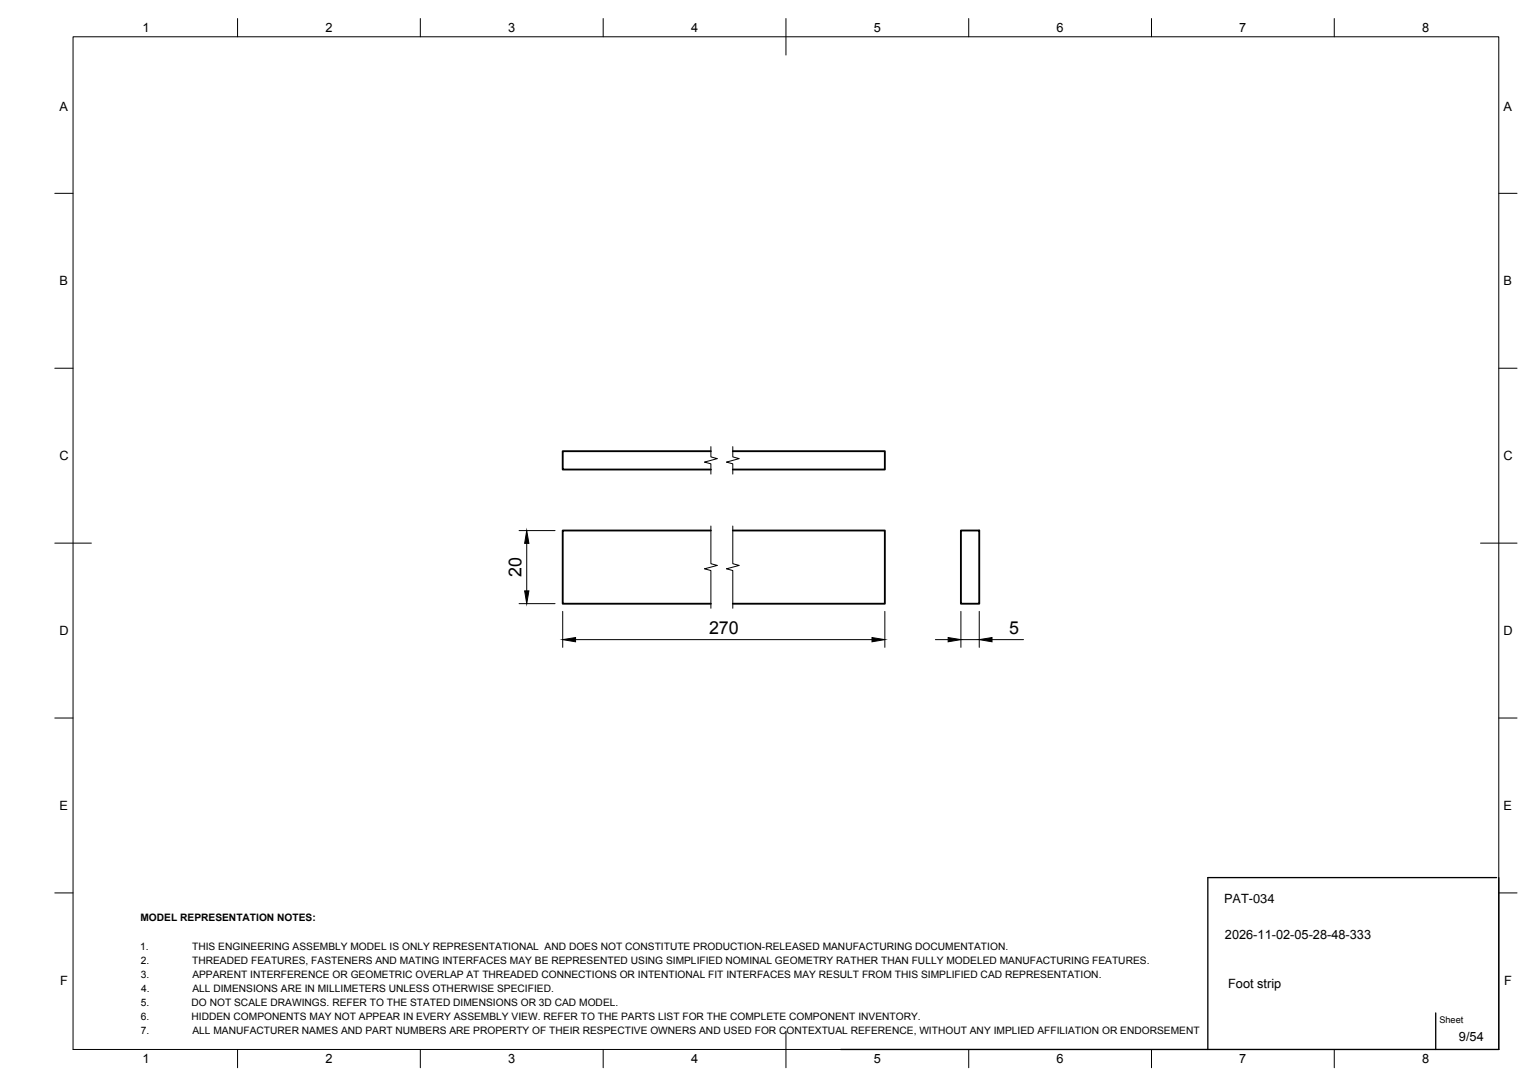
ISO-10303-21;
HEADER;
/* Generated by software containing ST-Developer
 * from STEP Tools, Inc. (www.steptools.com) 
 */

FILE_DESCRIPTION(
/* description */ ('Fatigue rig crank-slider'),
/* implementation_level */ '2;1');

FILE_NAME(
/* name */ 'Foot strip.step',
/* time_stamp */ '2026-10-28T03:24:50-07:00',
/* author */ (''),
/* organization */ (''),
/* preprocessor_version */ 'ST-DEVELOPER v20.2',
/* originating_system */ 'Autodesk Translation Framework v15.17.0.0',
/* authorisation */ '');

FILE_SCHEMA (('AUTOMOTIVE_DESIGN { 1 0 10303 214 3 1 1 }'));
ENDSEC;

DATA;
#10=MECHANICAL_DESIGN_GEOMETRIC_PRESENTATION_REPRESENTATION('',(#595),#16911);
#495=SHAPE_REPRESENTATION_RELATIONSHIP('SRR','None',#17134,#545);
#545=ADVANCED_BREP_SHAPE_REPRESENTATION('',(#654),#16863);
#595=STYLED_ITEM('',(#17473),#654);
#654=MANIFOLD_SOLID_BREP('Body1',#8886);
#949=PLANE('',#9712);
#950=PLANE('',#9713);
#951=PLANE('',#9714);
#952=PLANE('',#9715);
#953=PLANE('',#9716);
#954=PLANE('',#9717);
#1321=FACE_OUTER_BOUND('',#1920,.T.);
#1322=FACE_OUTER_BOUND('',#1921,.T.);
#1323=FACE_OUTER_BOUND('',#1922,.T.);
#1324=FACE_OUTER_BOUND('',#1923,.T.);
#1325=FACE_OUTER_BOUND('',#1924,.T.);
#1326=FACE_OUTER_BOUND('',#1925,.T.);
#1920=EDGE_LOOP('',(#6404,#6405,#6406,#6407));
#1921=EDGE_LOOP('',(#6408,#6409,#6410,#6411));
#1922=EDGE_LOOP('',(#6412,#6413,#6414,#6415));
#1923=EDGE_LOOP('',(#6416,#6417,#6418,#6419));
#1924=EDGE_LOOP('',(#6420,#6421,#6422,#6423));
#1925=EDGE_LOOP('',(#6424,#6425,#6426,#6427));
#2560=LINE('',#13816,#3206);
#2561=LINE('',#13818,#3207);
#2562=LINE('',#13820,#3208);
#2563=LINE('',#13821,#3209);
#2564=LINE('',#13824,#3210);
#2565=LINE('',#13826,#3211);
#2566=LINE('',#13827,#3212);
#2567=LINE('',#13830,#3213);
#2568=LINE('',#13832,#3214);
#2569=LINE('',#13833,#3215);
#2570=LINE('',#13835,#3216);
#2571=LINE('',#13836,#3217);
#3206=VECTOR('',#11106,1.);
#3207=VECTOR('',#11107,1.);
#3208=VECTOR('',#11108,1.);
#3209=VECTOR('',#11109,1.);
#3210=VECTOR('',#11112,1.);
#3211=VECTOR('',#11113,1.);
#3212=VECTOR('',#11114,1.);
#3213=VECTOR('',#11117,1.);
#3214=VECTOR('',#11118,1.);
#3215=VECTOR('',#11119,1.);
#3216=VECTOR('',#11122,1.);
#3217=VECTOR('',#11123,1.);
#4288=VERTEX_POINT('',#13814);
#4289=VERTEX_POINT('',#13815);
#4290=VERTEX_POINT('',#13817);
#4291=VERTEX_POINT('',#13819);
#4292=VERTEX_POINT('',#13823);
#4293=VERTEX_POINT('',#13825);
#4294=VERTEX_POINT('',#13829);
#4295=VERTEX_POINT('',#13831);
#5100=EDGE_CURVE('',#4288,#4289,#2560,.T.);
#5101=EDGE_CURVE('',#4289,#4290,#2561,.T.);
#5102=EDGE_CURVE('',#4291,#4290,#2562,.T.);
#5103=EDGE_CURVE('',#4288,#4291,#2563,.T.);
#5104=EDGE_CURVE('',#4292,#4288,#2564,.T.);
#5105=EDGE_CURVE('',#4293,#4291,#2565,.T.);
#5106=EDGE_CURVE('',#4292,#4293,#2566,.T.);
#5107=EDGE_CURVE('',#4294,#4292,#2567,.T.);
#5108=EDGE_CURVE('',#4295,#4293,#2568,.T.);
#5109=EDGE_CURVE('',#4294,#4295,#2569,.T.);
#5110=EDGE_CURVE('',#4289,#4294,#2570,.T.);
#5111=EDGE_CURVE('',#4290,#4295,#2571,.T.);
#6404=ORIENTED_EDGE('',*,*,#5100,.T.);
#6405=ORIENTED_EDGE('',*,*,#5101,.T.);
#6406=ORIENTED_EDGE('',*,*,#5102,.F.);
#6407=ORIENTED_EDGE('',*,*,#5103,.F.);
#6408=ORIENTED_EDGE('',*,*,#5104,.T.);
#6409=ORIENTED_EDGE('',*,*,#5103,.T.);
#6410=ORIENTED_EDGE('',*,*,#5105,.F.);
#6411=ORIENTED_EDGE('',*,*,#5106,.F.);
#6412=ORIENTED_EDGE('',*,*,#5107,.T.);
#6413=ORIENTED_EDGE('',*,*,#5106,.T.);
#6414=ORIENTED_EDGE('',*,*,#5108,.F.);
#6415=ORIENTED_EDGE('',*,*,#5109,.F.);
#6416=ORIENTED_EDGE('',*,*,#5110,.T.);
#6417=ORIENTED_EDGE('',*,*,#5109,.T.);
#6418=ORIENTED_EDGE('',*,*,#5111,.F.);
#6419=ORIENTED_EDGE('',*,*,#5101,.F.);
#6420=ORIENTED_EDGE('',*,*,#5111,.T.);
#6421=ORIENTED_EDGE('',*,*,#5108,.T.);
#6422=ORIENTED_EDGE('',*,*,#5105,.T.);
#6423=ORIENTED_EDGE('',*,*,#5102,.T.);
#6424=ORIENTED_EDGE('',*,*,#5110,.F.);
#6425=ORIENTED_EDGE('',*,*,#5100,.F.);
#6426=ORIENTED_EDGE('',*,*,#5104,.F.);
#6427=ORIENTED_EDGE('',*,*,#5107,.F.);
#8459=ADVANCED_FACE('',(#1321),#949,.T.);
#8460=ADVANCED_FACE('',(#1322),#950,.T.);
#8461=ADVANCED_FACE('',(#1323),#951,.T.);
#8462=ADVANCED_FACE('',(#1324),#952,.T.);
#8463=ADVANCED_FACE('',(#1325),#953,.T.);
#8464=ADVANCED_FACE('',(#1326),#954,.F.);
#8886=CLOSED_SHELL('',(#8459,#8460,#8461,#8462,#8463,#8464));
#9711=AXIS2_PLACEMENT_3D('',#13812,#11102,#11103);
#9712=AXIS2_PLACEMENT_3D('',#13813,#11104,#11105);
#9713=AXIS2_PLACEMENT_3D('',#13822,#11110,#11111);
#9714=AXIS2_PLACEMENT_3D('',#13828,#11115,#11116);
#9715=AXIS2_PLACEMENT_3D('',#13834,#11120,#11121);
#9716=AXIS2_PLACEMENT_3D('',#13837,#11124,#11125);
#9717=AXIS2_PLACEMENT_3D('',#13838,#11126,#11127);
#11102=DIRECTION('axis',(0.,0.,1.));
#11103=DIRECTION('refdir',(1.,0.,0.));
#11104=DIRECTION('center_axis',(0.,1.,0.));
#11105=DIRECTION('ref_axis',(-1.,0.,0.));
#11106=DIRECTION('',(-1.,0.,0.));
#11107=DIRECTION('',(0.,0.,1.));
#11108=DIRECTION('',(-1.,0.,0.));
#11109=DIRECTION('',(0.,0.,1.));
#11110=DIRECTION('center_axis',(1.,0.,0.));
#11111=DIRECTION('ref_axis',(0.,1.,0.));
#11112=DIRECTION('',(0.,1.,0.));
#11113=DIRECTION('',(0.,1.,0.));
#11114=DIRECTION('',(0.,0.,1.));
#11115=DIRECTION('center_axis',(0.,-1.,0.));
#11116=DIRECTION('ref_axis',(1.,0.,0.));
#11117=DIRECTION('',(1.,0.,0.));
#11118=DIRECTION('',(1.,0.,0.));
#11119=DIRECTION('',(0.,0.,1.));
#11120=DIRECTION('center_axis',(-1.,0.,0.));
#11121=DIRECTION('ref_axis',(0.,-1.,0.));
#11122=DIRECTION('',(0.,-1.,0.));
#11123=DIRECTION('',(0.,-1.,0.));
#11124=DIRECTION('center_axis',(0.,0.,1.));
#11125=DIRECTION('ref_axis',(1.,0.,0.));
#11126=DIRECTION('center_axis',(0.,0.,1.));
#11127=DIRECTION('ref_axis',(1.,0.,0.));
#13812=CARTESIAN_POINT('',(0.,0.,0.));
#13813=CARTESIAN_POINT('Origin',(-6.,9.,-0.5));
#13814=CARTESIAN_POINT('',(-6.,9.,-0.5));
#13815=CARTESIAN_POINT('',(-8.,9.,-0.5));
#13816=CARTESIAN_POINT('',(-6.,9.,-0.5));
#13817=CARTESIAN_POINT('',(-8.,9.,0.));
#13818=CARTESIAN_POINT('',(-8.,9.,-0.5));
#13819=CARTESIAN_POINT('',(-6.,9.,0.));
#13820=CARTESIAN_POINT('',(-6.,9.,0.));
#13821=CARTESIAN_POINT('',(-6.,9.,-0.5));
#13822=CARTESIAN_POINT('Origin',(-6.,-18.,-0.5));
#13823=CARTESIAN_POINT('',(-6.,-18.,-0.5));
#13824=CARTESIAN_POINT('',(-6.,-18.,-0.5));
#13825=CARTESIAN_POINT('',(-6.,-18.,0.));
#13826=CARTESIAN_POINT('',(-6.,-18.,0.));
#13827=CARTESIAN_POINT('',(-6.,-18.,-0.5));
#13828=CARTESIAN_POINT('Origin',(-8.,-18.,-0.5));
#13829=CARTESIAN_POINT('',(-8.,-18.,-0.5));
#13830=CARTESIAN_POINT('',(-8.,-18.,-0.5));
#13831=CARTESIAN_POINT('',(-8.,-18.,0.));
#13832=CARTESIAN_POINT('',(-8.,-18.,0.));
#13833=CARTESIAN_POINT('',(-8.,-18.,-0.5));
#13834=CARTESIAN_POINT('Origin',(-8.,9.,-0.5));
#13835=CARTESIAN_POINT('',(-8.,9.,-0.5));
#13836=CARTESIAN_POINT('',(-8.,9.,0.));
#13837=CARTESIAN_POINT('Origin',(-7.,-4.5,0.));
#13838=CARTESIAN_POINT('Origin',(-7.,-4.5,-0.5));
#16804=UNCERTAINTY_MEASURE_WITH_UNIT(LENGTH_MEASURE(0.001),#16912,
'DISTANCE_ACCURACY_VALUE',
'Maximum model space distance between geometric entities at asserted c
onnectivities');
#16852=UNCERTAINTY_MEASURE_WITH_UNIT(LENGTH_MEASURE(0.001),#16912,
'DISTANCE_ACCURACY_VALUE',
'Maximum model space distance between geometric entities at asserted c
onnectivities');
#16863=(
GEOMETRIC_REPRESENTATION_CONTEXT(3)
GLOBAL_UNCERTAINTY_ASSIGNED_CONTEXT((#16804))
GLOBAL_UNIT_ASSIGNED_CONTEXT((#16912,#16914,#16915))
REPRESENTATION_CONTEXT('','3D')
);
#16911=(
GEOMETRIC_REPRESENTATION_CONTEXT(3)
GLOBAL_UNCERTAINTY_ASSIGNED_CONTEXT((#16852))
GLOBAL_UNIT_ASSIGNED_CONTEXT((#16912,#16914,#16915))
REPRESENTATION_CONTEXT('','3D')
);
#16912=(
LENGTH_UNIT()
NAMED_UNIT(*)
SI_UNIT(.CENTI.,.METRE.)
);
#16914=(
NAMED_UNIT(*)
PLANE_ANGLE_UNIT()
SI_UNIT($,.RADIAN.)
);
#16915=(
NAMED_UNIT(*)
SI_UNIT($,.STERADIAN.)
SOLID_ANGLE_UNIT()
);
#16926=SHAPE_DEFINITION_REPRESENTATION(#16984,#17134);
#16984=PRODUCT_DEFINITION_SHAPE('',$,#17193);
#17134=SHAPE_REPRESENTATION('',(#9711),#16863);
#17182=PRODUCT_DEFINITION_CONTEXT('part definition',#17358,'design');
#17193=PRODUCT_DEFINITION('Foot strip','Foot strip',#17251,#17182);
#17251=PRODUCT_DEFINITION_FORMATION('',$,#17370);
#17358=APPLICATION_CONTEXT(
'Core Data for Automotive Mechanical Design Process');
#17359=PRODUCT_CONTEXT('part definition',#17358,'mechanical');
#17370=PRODUCT('Foot strip','Foot strip','Foot strip',(#17359));
#17467=COLOUR_RGB('Light Blue',0.38,0.62,0.78);
#17468=FILL_AREA_STYLE_COLOUR('',#17467);
#17469=FILL_AREA_STYLE('',(#17468));
#17470=SURFACE_STYLE_FILL_AREA(#17469);
#17471=SURFACE_SIDE_STYLE('',(#17470));
#17472=SURFACE_STYLE_USAGE(.BOTH.,#17471);
#17473=PRESENTATION_STYLE_ASSIGNMENT((#17472));
ENDSEC;
END-ISO-10303-21;
